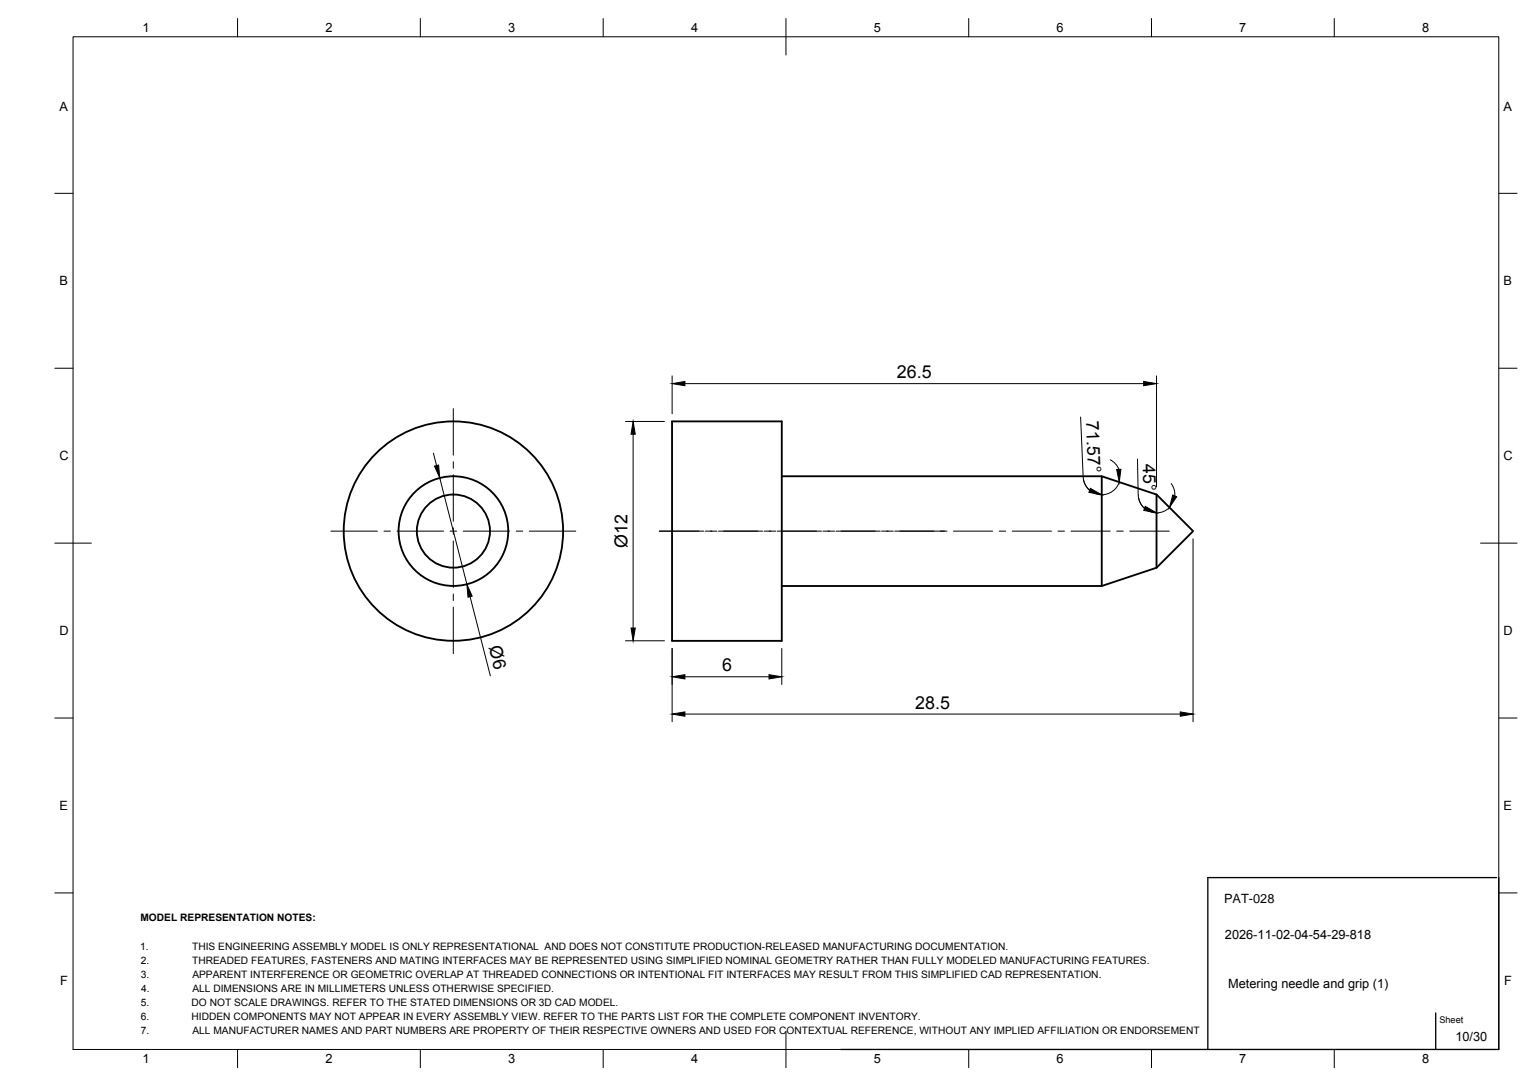
ISO-10303-21;
HEADER;
/* Generated by software containing ST-Developer
 * from STEP Tools, Inc. (www.steptools.com) 
 */

FILE_DESCRIPTION(
/* description */ ('Cylinder foot and clevis mount kit'),
/* implementation_level */ '2;1');

FILE_NAME(
/* name */ 'Metering needle and grip (1).step',
/* time_stamp */ '2026-10-27T20:10:43-07:00',
/* author */ (''),
/* organization */ (''),
/* preprocessor_version */ 'ST-DEVELOPER v20.2',
/* originating_system */ 'Autodesk Translation Framework v15.17.0.0',
/* authorisation */ '');

FILE_SCHEMA (('AUTOMOTIVE_DESIGN { 1 0 10303 214 3 1 1 }'));
ENDSEC;

DATA;
#10=MECHANICAL_DESIGN_GEOMETRIC_PRESENTATION_REPRESENTATION('',(#343),#9102);
#265=CONICAL_SURFACE('',#5503,0.1,0.78539816339745);
#266=CONICAL_SURFACE('',#5505,0.25,0.321750554396641);
#287=SHAPE_REPRESENTATION_RELATIONSHIP('SRR','None',#9234,#315);
#315=ADVANCED_BREP_SHAPE_REPRESENTATION('',(#371),#9077);
#343=STYLED_ITEM('',(#9467),#371);
#371=MANIFOLD_SOLID_BREP('Body1',#4929);
#439=FACE_BOUND('',#1179,.T.);
#589=PLANE('',#5509);
#590=PLANE('',#5513);
#822=FACE_OUTER_BOUND('',#1175,.T.);
#823=FACE_OUTER_BOUND('',#1176,.T.);
#824=FACE_OUTER_BOUND('',#1177,.T.);
#825=FACE_OUTER_BOUND('',#1178,.T.);
#826=FACE_OUTER_BOUND('',#1180,.T.);
#827=FACE_OUTER_BOUND('',#1181,.T.);
#1175=EDGE_LOOP('',(#3843,#3844,#3845));
#1176=EDGE_LOOP('',(#3846,#3847,#3848,#3849));
#1177=EDGE_LOOP('',(#3850,#3851,#3852,#3853));
#1178=EDGE_LOOP('',(#3854));
#1179=EDGE_LOOP('',(#3855));
#1180=EDGE_LOOP('',(#3856,#3857,#3858,#3859));
#1181=EDGE_LOOP('',(#3860));
#1569=LINE('',#8063,#1918);
#1570=LINE('',#8067,#1919);
#1571=LINE('',#8071,#1920);
#1572=LINE('',#8078,#1921);
#1918=VECTOR('',#6534,0.1);
#1919=VECTOR('',#6539,0.25);
#1920=VECTOR('',#6544,0.3);
#1921=VECTOR('',#6553,0.6);
#2199=CIRCLE('',#5504,0.2);
#2200=CIRCLE('',#5506,0.3);
#2201=CIRCLE('',#5508,0.3);
#2202=CIRCLE('',#5510,0.6);
#2203=CIRCLE('',#5512,0.6);
#2492=VERTEX_POINT('',#8060);
#2493=VERTEX_POINT('',#8062);
#2494=VERTEX_POINT('',#8065);
#2495=VERTEX_POINT('',#8069);
#2496=VERTEX_POINT('',#8073);
#2497=VERTEX_POINT('',#8076);
#2976=EDGE_CURVE('',#2492,#2492,#2199,.T.);
#2977=EDGE_CURVE('',#2492,#2493,#1569,.T.);
#2978=EDGE_CURVE('',#2494,#2494,#2200,.T.);
#2979=EDGE_CURVE('',#2494,#2492,#1570,.T.);
#2980=EDGE_CURVE('',#2495,#2495,#2201,.T.);
#2981=EDGE_CURVE('',#2495,#2494,#1571,.T.);
#2982=EDGE_CURVE('',#2496,#2496,#2202,.T.);
#2983=EDGE_CURVE('',#2497,#2497,#2203,.T.);
#2984=EDGE_CURVE('',#2497,#2496,#1572,.T.);
#3843=ORIENTED_EDGE('',*,*,#2976,.F.);
#3844=ORIENTED_EDGE('',*,*,#2977,.T.);
#3845=ORIENTED_EDGE('',*,*,#2977,.F.);
#3846=ORIENTED_EDGE('',*,*,#2978,.F.);
#3847=ORIENTED_EDGE('',*,*,#2979,.T.);
#3848=ORIENTED_EDGE('',*,*,#2976,.T.);
#3849=ORIENTED_EDGE('',*,*,#2979,.F.);
#3850=ORIENTED_EDGE('',*,*,#2980,.F.);
#3851=ORIENTED_EDGE('',*,*,#2981,.T.);
#3852=ORIENTED_EDGE('',*,*,#2978,.T.);
#3853=ORIENTED_EDGE('',*,*,#2981,.F.);
#3854=ORIENTED_EDGE('',*,*,#2982,.F.);
#3855=ORIENTED_EDGE('',*,*,#2980,.T.);
#3856=ORIENTED_EDGE('',*,*,#2983,.F.);
#3857=ORIENTED_EDGE('',*,*,#2984,.T.);
#3858=ORIENTED_EDGE('',*,*,#2982,.T.);
#3859=ORIENTED_EDGE('',*,*,#2984,.F.);
#3860=ORIENTED_EDGE('',*,*,#2983,.T.);
#4566=CYLINDRICAL_SURFACE('',#5507,0.3);
#4567=CYLINDRICAL_SURFACE('',#5511,0.6);
#4745=ADVANCED_FACE('',(#822),#265,.T.);
#4746=ADVANCED_FACE('',(#823),#266,.T.);
#4747=ADVANCED_FACE('',(#824),#4566,.T.);
#4748=ADVANCED_FACE('',(#825,#439),#589,.T.);
#4749=ADVANCED_FACE('',(#826),#4567,.T.);
#4750=ADVANCED_FACE('',(#827),#590,.T.);
#4929=CLOSED_SHELL('',(#4745,#4746,#4747,#4748,#4749,#4750));
#5502=AXIS2_PLACEMENT_3D('',#8058,#6528,#6529);
#5503=AXIS2_PLACEMENT_3D('',#8059,#6530,#6531);
#5504=AXIS2_PLACEMENT_3D('',#8061,#6532,#6533);
#5505=AXIS2_PLACEMENT_3D('',#8064,#6535,#6536);
#5506=AXIS2_PLACEMENT_3D('',#8066,#6537,#6538);
#5507=AXIS2_PLACEMENT_3D('',#8068,#6540,#6541);
#5508=AXIS2_PLACEMENT_3D('',#8070,#6542,#6543);
#5509=AXIS2_PLACEMENT_3D('',#8072,#6545,#6546);
#5510=AXIS2_PLACEMENT_3D('',#8074,#6547,#6548);
#5511=AXIS2_PLACEMENT_3D('',#8075,#6549,#6550);
#5512=AXIS2_PLACEMENT_3D('',#8077,#6551,#6552);
#5513=AXIS2_PLACEMENT_3D('',#8079,#6554,#6555);
#6528=DIRECTION('axis',(0.,0.,1.));
#6529=DIRECTION('refdir',(1.,0.,0.));
#6530=DIRECTION('center_axis',(0.,0.,1.));
#6531=DIRECTION('ref_axis',(1.,0.,0.));
#6532=DIRECTION('center_axis',(0.,0.,1.));
#6533=DIRECTION('ref_axis',(1.,0.,0.));
#6534=DIRECTION('',(0.707106781186549,8.65956056235495E-17,-0.707106781186546));
#6535=DIRECTION('center_axis',(0.,0.,1.));
#6536=DIRECTION('ref_axis',(1.,0.,0.));
#6537=DIRECTION('center_axis',(0.,0.,1.));
#6538=DIRECTION('ref_axis',(1.,0.,0.));
#6539=DIRECTION('',(0.316227766016837,3.87267321454038E-17,-0.948683298050514));
#6540=DIRECTION('center_axis',(0.,0.,1.));
#6541=DIRECTION('ref_axis',(1.,0.,0.));
#6542=DIRECTION('center_axis',(0.,0.,1.));
#6543=DIRECTION('ref_axis',(1.,0.,0.));
#6544=DIRECTION('',(0.,0.,-1.));
#6545=DIRECTION('center_axis',(0.,0.,-1.));
#6546=DIRECTION('ref_axis',(-1.,0.,0.));
#6547=DIRECTION('center_axis',(0.,0.,1.));
#6548=DIRECTION('ref_axis',(1.,0.,0.));
#6549=DIRECTION('center_axis',(0.,0.,1.));
#6550=DIRECTION('ref_axis',(1.,0.,0.));
#6551=DIRECTION('center_axis',(0.,0.,1.));
#6552=DIRECTION('ref_axis',(1.,0.,0.));
#6553=DIRECTION('',(0.,0.,-1.));
#6554=DIRECTION('center_axis',(0.,0.,1.));
#6555=DIRECTION('ref_axis',(1.,0.,0.));
#8058=CARTESIAN_POINT('',(0.,0.,0.));
#8059=CARTESIAN_POINT('Origin',(0.,11.8,8.15));
#8060=CARTESIAN_POINT('',(-0.2,11.8,8.25));
#8061=CARTESIAN_POINT('Origin',(0.,11.8,8.25));
#8062=CARTESIAN_POINT('',(0.,11.8,8.05));
#8063=CARTESIAN_POINT('',(-0.1,11.8,8.15));
#8064=CARTESIAN_POINT('Origin',(0.,11.8,8.4));
#8065=CARTESIAN_POINT('',(-0.3,11.8,8.55));
#8066=CARTESIAN_POINT('Origin',(0.,11.8,8.55));
#8067=CARTESIAN_POINT('',(-0.25,11.8,8.4));
#8068=CARTESIAN_POINT('Origin',(0.,11.8,9.425));
#8069=CARTESIAN_POINT('',(-0.3,11.8,10.3));
#8070=CARTESIAN_POINT('Origin',(0.,11.8,10.3));
#8071=CARTESIAN_POINT('',(-0.3,11.8,9.425));
#8072=CARTESIAN_POINT('Origin',(0.6,11.8,10.3));
#8073=CARTESIAN_POINT('',(-0.6,11.8,10.3));
#8074=CARTESIAN_POINT('Origin',(0.,11.8,10.3));
#8075=CARTESIAN_POINT('Origin',(0.,11.8,10.6));
#8076=CARTESIAN_POINT('',(-0.6,11.8,10.9));
#8077=CARTESIAN_POINT('Origin',(0.,11.8,10.9));
#8078=CARTESIAN_POINT('',(-0.6,11.8,10.6));
#8079=CARTESIAN_POINT('Origin',(0.,11.8,10.9));
#9044=UNCERTAINTY_MEASURE_WITH_UNIT(LENGTH_MEASURE(0.001),#9103,
'DISTANCE_ACCURACY_VALUE',
'Maximum model space distance between geometric entities at asserted c
onnectivities');
#9069=UNCERTAINTY_MEASURE_WITH_UNIT(LENGTH_MEASURE(0.001),#9103,
'DISTANCE_ACCURACY_VALUE',
'Maximum model space distance between geometric entities at asserted c
onnectivities');
#9077=(
GEOMETRIC_REPRESENTATION_CONTEXT(3)
GLOBAL_UNCERTAINTY_ASSIGNED_CONTEXT((#9044))
GLOBAL_UNIT_ASSIGNED_CONTEXT((#9103,#9105,#9106))
REPRESENTATION_CONTEXT('','3D')
);
#9102=(
GEOMETRIC_REPRESENTATION_CONTEXT(3)
GLOBAL_UNCERTAINTY_ASSIGNED_CONTEXT((#9069))
GLOBAL_UNIT_ASSIGNED_CONTEXT((#9103,#9105,#9106))
REPRESENTATION_CONTEXT('','3D')
);
#9103=(
LENGTH_UNIT()
NAMED_UNIT(*)
SI_UNIT(.CENTI.,.METRE.)
);
#9105=(
NAMED_UNIT(*)
PLANE_ANGLE_UNIT()
SI_UNIT($,.RADIAN.)
);
#9106=(
NAMED_UNIT(*)
SI_UNIT($,.STERADIAN.)
SOLID_ANGLE_UNIT()
);
#9114=SHAPE_DEFINITION_REPRESENTATION(#9146,#9234);
#9146=PRODUCT_DEFINITION_SHAPE('',$,#9267);
#9234=SHAPE_REPRESENTATION('',(#5502),#9077);
#9259=PRODUCT_DEFINITION_CONTEXT('part definition',#9357,'design');
#9267=PRODUCT_DEFINITION('Metering needle and grip (1)',
'Metering needle and grip (1)',#9299,#9259);
#9299=PRODUCT_DEFINITION_FORMATION('',$,#9366);
#9357=APPLICATION_CONTEXT(
'Core Data for Automotive Mechanical Design Process');
#9358=PRODUCT_CONTEXT('part definition',#9357,'mechanical');
#9366=PRODUCT('Metering needle and grip (1)',
'Metering needle and grip (1)','Metering needle and grip (1)',(#9358));
#9461=COLOUR_RGB('Black',0.12,0.14,0.17);
#9462=FILL_AREA_STYLE_COLOUR('',#9461);
#9463=FILL_AREA_STYLE('',(#9462));
#9464=SURFACE_STYLE_FILL_AREA(#9463);
#9465=SURFACE_SIDE_STYLE('',(#9464));
#9466=SURFACE_STYLE_USAGE(.BOTH.,#9465);
#9467=PRESENTATION_STYLE_ASSIGNMENT((#9466));
ENDSEC;
END-ISO-10303-21;
